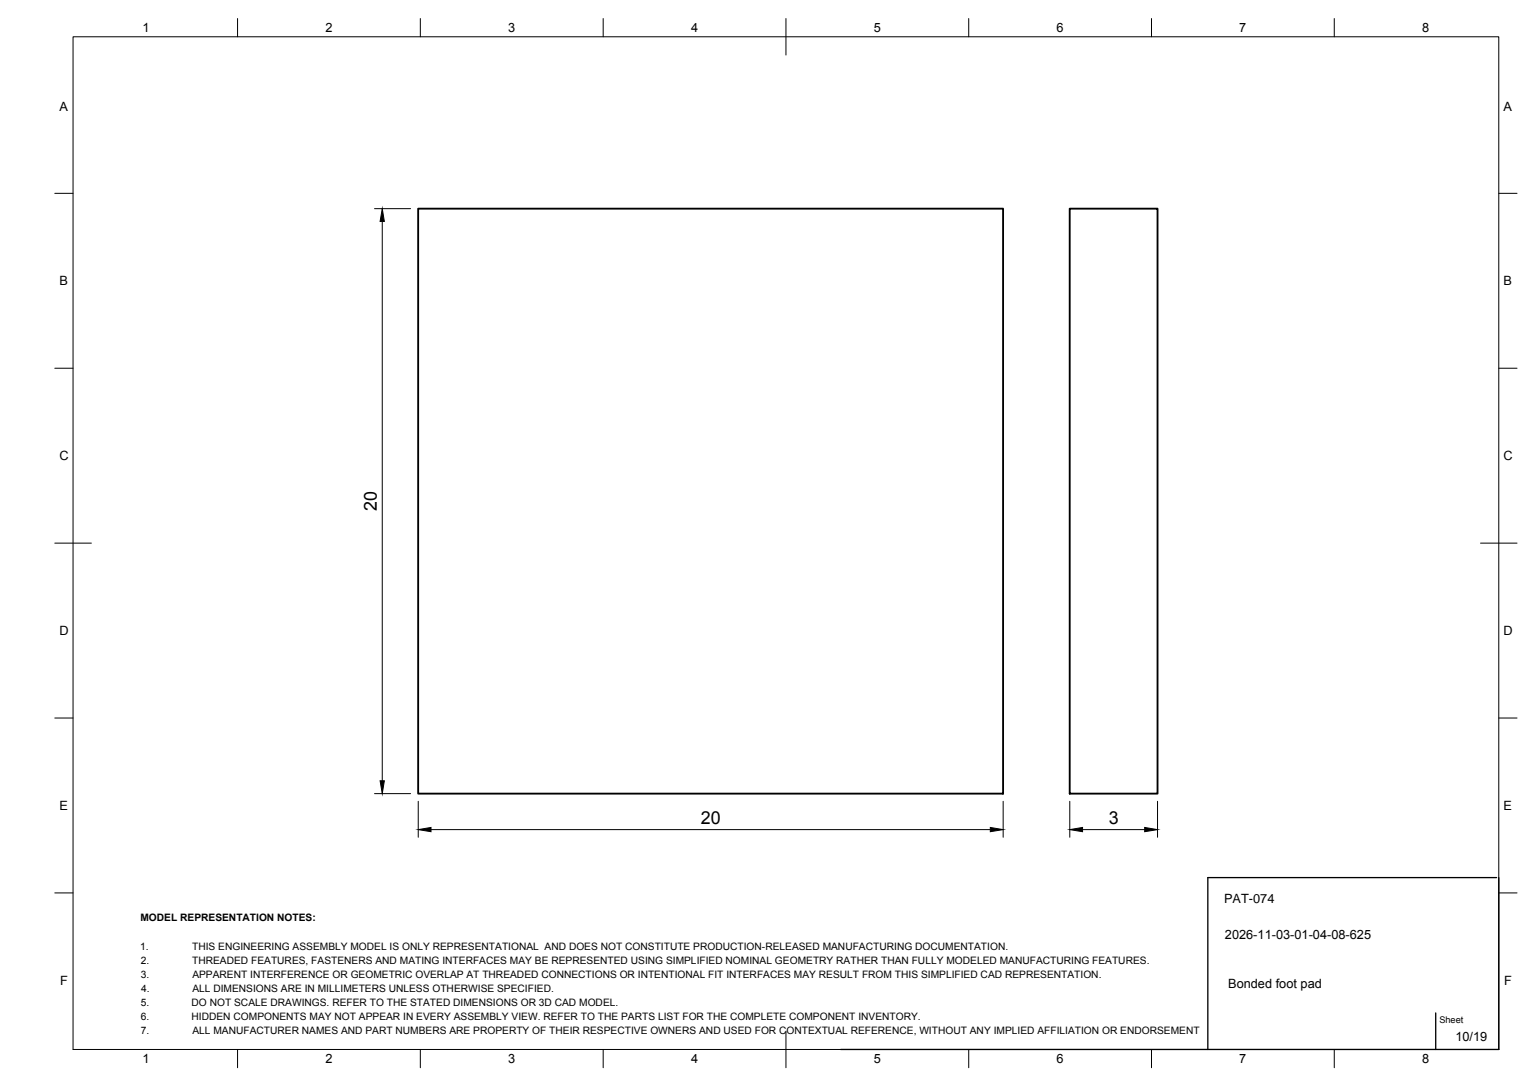
ISO-10303-21;
HEADER;
/* Generated by software containing ST-Developer
 * from STEP Tools, Inc. (www.steptools.com) 
 */

FILE_DESCRIPTION(
/* description */ ('Manual rail carriage with stops'),
/* implementation_level */ '2;1');

FILE_NAME(
/* name */ 'Bonded foot pad.step',
/* time_stamp */ '2026-10-27T18:54:27-07:00',
/* author */ (''),
/* organization */ (''),
/* preprocessor_version */ 'ST-DEVELOPER v20.2',
/* originating_system */ 'Autodesk Translation Framework v15.17.0.0',
/* authorisation */ '');

FILE_SCHEMA (('AUTOMOTIVE_DESIGN { 1 0 10303 214 3 1 1 }'));
ENDSEC;

DATA;
#10=MECHANICAL_DESIGN_GEOMETRIC_PRESENTATION_REPRESENTATION('',(#281),#8499);
#245=SHAPE_REPRESENTATION_RELATIONSHIP('SRR','None',#8608,#263);
#263=ADVANCED_BREP_SHAPE_REPRESENTATION('',(#297),#8487);
#281=STYLED_ITEM('',(#8781),#297);
#297=MANIFOLD_SOLID_BREP('Body1',#4951);
#499=PLANE('',#5406);
#500=PLANE('',#5407);
#501=PLANE('',#5408);
#502=PLANE('',#5409);
#503=PLANE('',#5410);
#504=PLANE('',#5411);
#735=FACE_OUTER_BOUND('',#1051,.T.);
#736=FACE_OUTER_BOUND('',#1052,.T.);
#737=FACE_OUTER_BOUND('',#1053,.T.);
#738=FACE_OUTER_BOUND('',#1054,.T.);
#739=FACE_OUTER_BOUND('',#1055,.T.);
#740=FACE_OUTER_BOUND('',#1056,.T.);
#1051=EDGE_LOOP('',(#4132,#4133,#4134,#4135));
#1052=EDGE_LOOP('',(#4136,#4137,#4138,#4139));
#1053=EDGE_LOOP('',(#4140,#4141,#4142,#4143));
#1054=EDGE_LOOP('',(#4144,#4145,#4146,#4147));
#1055=EDGE_LOOP('',(#4148,#4149,#4150,#4151));
#1056=EDGE_LOOP('',(#4152,#4153,#4154,#4155));
#1493=LINE('',#7882,#1993);
#1494=LINE('',#7884,#1994);
#1495=LINE('',#7886,#1995);
#1496=LINE('',#7887,#1996);
#1497=LINE('',#7890,#1997);
#1498=LINE('',#7892,#1998);
#1499=LINE('',#7893,#1999);
#1500=LINE('',#7896,#2000);
#1501=LINE('',#7898,#2001);
#1502=LINE('',#7899,#2002);
#1503=LINE('',#7901,#2003);
#1504=LINE('',#7902,#2004);
#1993=VECTOR('',#6432,1.);
#1994=VECTOR('',#6433,1.);
#1995=VECTOR('',#6434,1.);
#1996=VECTOR('',#6435,1.);
#1997=VECTOR('',#6438,1.);
#1998=VECTOR('',#6439,1.);
#1999=VECTOR('',#6440,1.);
#2000=VECTOR('',#6443,1.);
#2001=VECTOR('',#6444,1.);
#2002=VECTOR('',#6445,1.);
#2003=VECTOR('',#6448,1.);
#2004=VECTOR('',#6449,1.);
#2567=VERTEX_POINT('',#7880);
#2568=VERTEX_POINT('',#7881);
#2569=VERTEX_POINT('',#7883);
#2570=VERTEX_POINT('',#7885);
#2571=VERTEX_POINT('',#7889);
#2572=VERTEX_POINT('',#7891);
#2573=VERTEX_POINT('',#7895);
#2574=VERTEX_POINT('',#7897);
#3114=EDGE_CURVE('',#2567,#2568,#1493,.T.);
#3115=EDGE_CURVE('',#2568,#2569,#1494,.T.);
#3116=EDGE_CURVE('',#2570,#2569,#1495,.T.);
#3117=EDGE_CURVE('',#2567,#2570,#1496,.T.);
#3118=EDGE_CURVE('',#2571,#2567,#1497,.T.);
#3119=EDGE_CURVE('',#2572,#2570,#1498,.T.);
#3120=EDGE_CURVE('',#2571,#2572,#1499,.T.);
#3121=EDGE_CURVE('',#2573,#2571,#1500,.T.);
#3122=EDGE_CURVE('',#2574,#2572,#1501,.T.);
#3123=EDGE_CURVE('',#2573,#2574,#1502,.T.);
#3124=EDGE_CURVE('',#2568,#2573,#1503,.T.);
#3125=EDGE_CURVE('',#2569,#2574,#1504,.T.);
#4132=ORIENTED_EDGE('',*,*,#3114,.T.);
#4133=ORIENTED_EDGE('',*,*,#3115,.T.);
#4134=ORIENTED_EDGE('',*,*,#3116,.F.);
#4135=ORIENTED_EDGE('',*,*,#3117,.F.);
#4136=ORIENTED_EDGE('',*,*,#3118,.T.);
#4137=ORIENTED_EDGE('',*,*,#3117,.T.);
#4138=ORIENTED_EDGE('',*,*,#3119,.F.);
#4139=ORIENTED_EDGE('',*,*,#3120,.F.);
#4140=ORIENTED_EDGE('',*,*,#3121,.T.);
#4141=ORIENTED_EDGE('',*,*,#3120,.T.);
#4142=ORIENTED_EDGE('',*,*,#3122,.F.);
#4143=ORIENTED_EDGE('',*,*,#3123,.F.);
#4144=ORIENTED_EDGE('',*,*,#3124,.T.);
#4145=ORIENTED_EDGE('',*,*,#3123,.T.);
#4146=ORIENTED_EDGE('',*,*,#3125,.F.);
#4147=ORIENTED_EDGE('',*,*,#3115,.F.);
#4148=ORIENTED_EDGE('',*,*,#3125,.T.);
#4149=ORIENTED_EDGE('',*,*,#3122,.T.);
#4150=ORIENTED_EDGE('',*,*,#3119,.T.);
#4151=ORIENTED_EDGE('',*,*,#3116,.T.);
#4152=ORIENTED_EDGE('',*,*,#3124,.F.);
#4153=ORIENTED_EDGE('',*,*,#3114,.F.);
#4154=ORIENTED_EDGE('',*,*,#3118,.F.);
#4155=ORIENTED_EDGE('',*,*,#3121,.F.);
#4834=ADVANCED_FACE('',(#735),#499,.T.);
#4835=ADVANCED_FACE('',(#736),#500,.T.);
#4836=ADVANCED_FACE('',(#737),#501,.T.);
#4837=ADVANCED_FACE('',(#738),#502,.T.);
#4838=ADVANCED_FACE('',(#739),#503,.T.);
#4839=ADVANCED_FACE('',(#740),#504,.F.);
#4951=CLOSED_SHELL('',(#4834,#4835,#4836,#4837,#4838,#4839));
#5405=AXIS2_PLACEMENT_3D('',#7878,#6428,#6429);
#5406=AXIS2_PLACEMENT_3D('',#7879,#6430,#6431);
#5407=AXIS2_PLACEMENT_3D('',#7888,#6436,#6437);
#5408=AXIS2_PLACEMENT_3D('',#7894,#6441,#6442);
#5409=AXIS2_PLACEMENT_3D('',#7900,#6446,#6447);
#5410=AXIS2_PLACEMENT_3D('',#7903,#6450,#6451);
#5411=AXIS2_PLACEMENT_3D('',#7904,#6452,#6453);
#6428=DIRECTION('axis',(0.,0.,1.));
#6429=DIRECTION('refdir',(1.,0.,0.));
#6430=DIRECTION('center_axis',(0.,1.,0.));
#6431=DIRECTION('ref_axis',(-1.,0.,0.));
#6432=DIRECTION('',(-1.,0.,0.));
#6433=DIRECTION('',(0.,0.,1.));
#6434=DIRECTION('',(-1.,0.,0.));
#6435=DIRECTION('',(0.,0.,1.));
#6436=DIRECTION('center_axis',(1.,0.,0.));
#6437=DIRECTION('ref_axis',(0.,1.,0.));
#6438=DIRECTION('',(0.,1.,0.));
#6439=DIRECTION('',(0.,1.,0.));
#6440=DIRECTION('',(0.,0.,1.));
#6441=DIRECTION('center_axis',(0.,-1.,0.));
#6442=DIRECTION('ref_axis',(1.,0.,0.));
#6443=DIRECTION('',(1.,0.,0.));
#6444=DIRECTION('',(1.,0.,0.));
#6445=DIRECTION('',(0.,0.,1.));
#6446=DIRECTION('center_axis',(-1.,0.,0.));
#6447=DIRECTION('ref_axis',(0.,-1.,0.));
#6448=DIRECTION('',(0.,-1.,0.));
#6449=DIRECTION('',(0.,-1.,0.));
#6450=DIRECTION('center_axis',(0.,0.,1.));
#6451=DIRECTION('ref_axis',(1.,0.,0.));
#6452=DIRECTION('center_axis',(0.,0.,1.));
#6453=DIRECTION('ref_axis',(1.,0.,0.));
#7878=CARTESIAN_POINT('',(0.,0.,0.));
#7879=CARTESIAN_POINT('Origin',(4.,-2.5,-0.3));
#7880=CARTESIAN_POINT('',(4.,-2.5,-0.3));
#7881=CARTESIAN_POINT('',(2.,-2.5,-0.3));
#7882=CARTESIAN_POINT('',(4.,-2.5,-0.3));
#7883=CARTESIAN_POINT('',(2.,-2.5,0.));
#7884=CARTESIAN_POINT('',(2.,-2.5,-0.3));
#7885=CARTESIAN_POINT('',(4.,-2.5,0.));
#7886=CARTESIAN_POINT('',(4.,-2.5,0.));
#7887=CARTESIAN_POINT('',(4.,-2.5,-0.3));
#7888=CARTESIAN_POINT('Origin',(4.,-4.5,-0.3));
#7889=CARTESIAN_POINT('',(4.,-4.5,-0.3));
#7890=CARTESIAN_POINT('',(4.,-4.5,-0.3));
#7891=CARTESIAN_POINT('',(4.,-4.5,0.));
#7892=CARTESIAN_POINT('',(4.,-4.5,0.));
#7893=CARTESIAN_POINT('',(4.,-4.5,-0.3));
#7894=CARTESIAN_POINT('Origin',(2.,-4.5,-0.3));
#7895=CARTESIAN_POINT('',(2.,-4.5,-0.3));
#7896=CARTESIAN_POINT('',(2.,-4.5,-0.3));
#7897=CARTESIAN_POINT('',(2.,-4.5,0.));
#7898=CARTESIAN_POINT('',(2.,-4.5,0.));
#7899=CARTESIAN_POINT('',(2.,-4.5,-0.3));
#7900=CARTESIAN_POINT('Origin',(2.,-2.5,-0.3));
#7901=CARTESIAN_POINT('',(2.,-2.5,-0.3));
#7902=CARTESIAN_POINT('',(2.,-2.5,0.));
#7903=CARTESIAN_POINT('Origin',(3.,-3.5,0.));
#7904=CARTESIAN_POINT('Origin',(3.,-3.5,-0.3));
#8464=UNCERTAINTY_MEASURE_WITH_UNIT(LENGTH_MEASURE(0.001),#8500,
'DISTANCE_ACCURACY_VALUE',
'Maximum model space distance between geometric entities at asserted c
onnectivities');
#8476=UNCERTAINTY_MEASURE_WITH_UNIT(LENGTH_MEASURE(0.001),#8500,
'DISTANCE_ACCURACY_VALUE',
'Maximum model space distance between geometric entities at asserted c
onnectivities');
#8487=(
GEOMETRIC_REPRESENTATION_CONTEXT(3)
GLOBAL_UNCERTAINTY_ASSIGNED_CONTEXT((#8464))
GLOBAL_UNIT_ASSIGNED_CONTEXT((#8500,#8502,#8503))
REPRESENTATION_CONTEXT('','3D')
);
#8499=(
GEOMETRIC_REPRESENTATION_CONTEXT(3)
GLOBAL_UNCERTAINTY_ASSIGNED_CONTEXT((#8476))
GLOBAL_UNIT_ASSIGNED_CONTEXT((#8500,#8502,#8503))
REPRESENTATION_CONTEXT('','3D')
);
#8500=(
LENGTH_UNIT()
NAMED_UNIT(*)
SI_UNIT(.CENTI.,.METRE.)
);
#8502=(
NAMED_UNIT(*)
PLANE_ANGLE_UNIT()
SI_UNIT($,.RADIAN.)
);
#8503=(
NAMED_UNIT(*)
SI_UNIT($,.STERADIAN.)
SOLID_ANGLE_UNIT()
);
#8514=SHAPE_DEFINITION_REPRESENTATION(#8536,#8608);
#8536=PRODUCT_DEFINITION_SHAPE('',$,#8631);
#8608=SHAPE_REPRESENTATION('',(#5405),#8487);
#8620=PRODUCT_DEFINITION_CONTEXT('part definition',#8688,'design');
#8631=PRODUCT_DEFINITION('Bonded foot pad','Bonded foot pad',#8653,#8620);
#8653=PRODUCT_DEFINITION_FORMATION('',$,#8700);
#8688=APPLICATION_CONTEXT(
'Core Data for Automotive Mechanical Design Process');
#8689=PRODUCT_CONTEXT('part definition',#8688,'mechanical');
#8700=PRODUCT('Bonded foot pad','Bonded foot pad','Bonded foot pad',(#8689));
#8775=COLOUR_RGB('Sky Blue',0.24,0.69,0.87);
#8776=FILL_AREA_STYLE_COLOUR('',#8775);
#8777=FILL_AREA_STYLE('',(#8776));
#8778=SURFACE_STYLE_FILL_AREA(#8777);
#8779=SURFACE_SIDE_STYLE('',(#8778));
#8780=SURFACE_STYLE_USAGE(.BOTH.,#8779);
#8781=PRESENTATION_STYLE_ASSIGNMENT((#8780));
ENDSEC;
END-ISO-10303-21;
